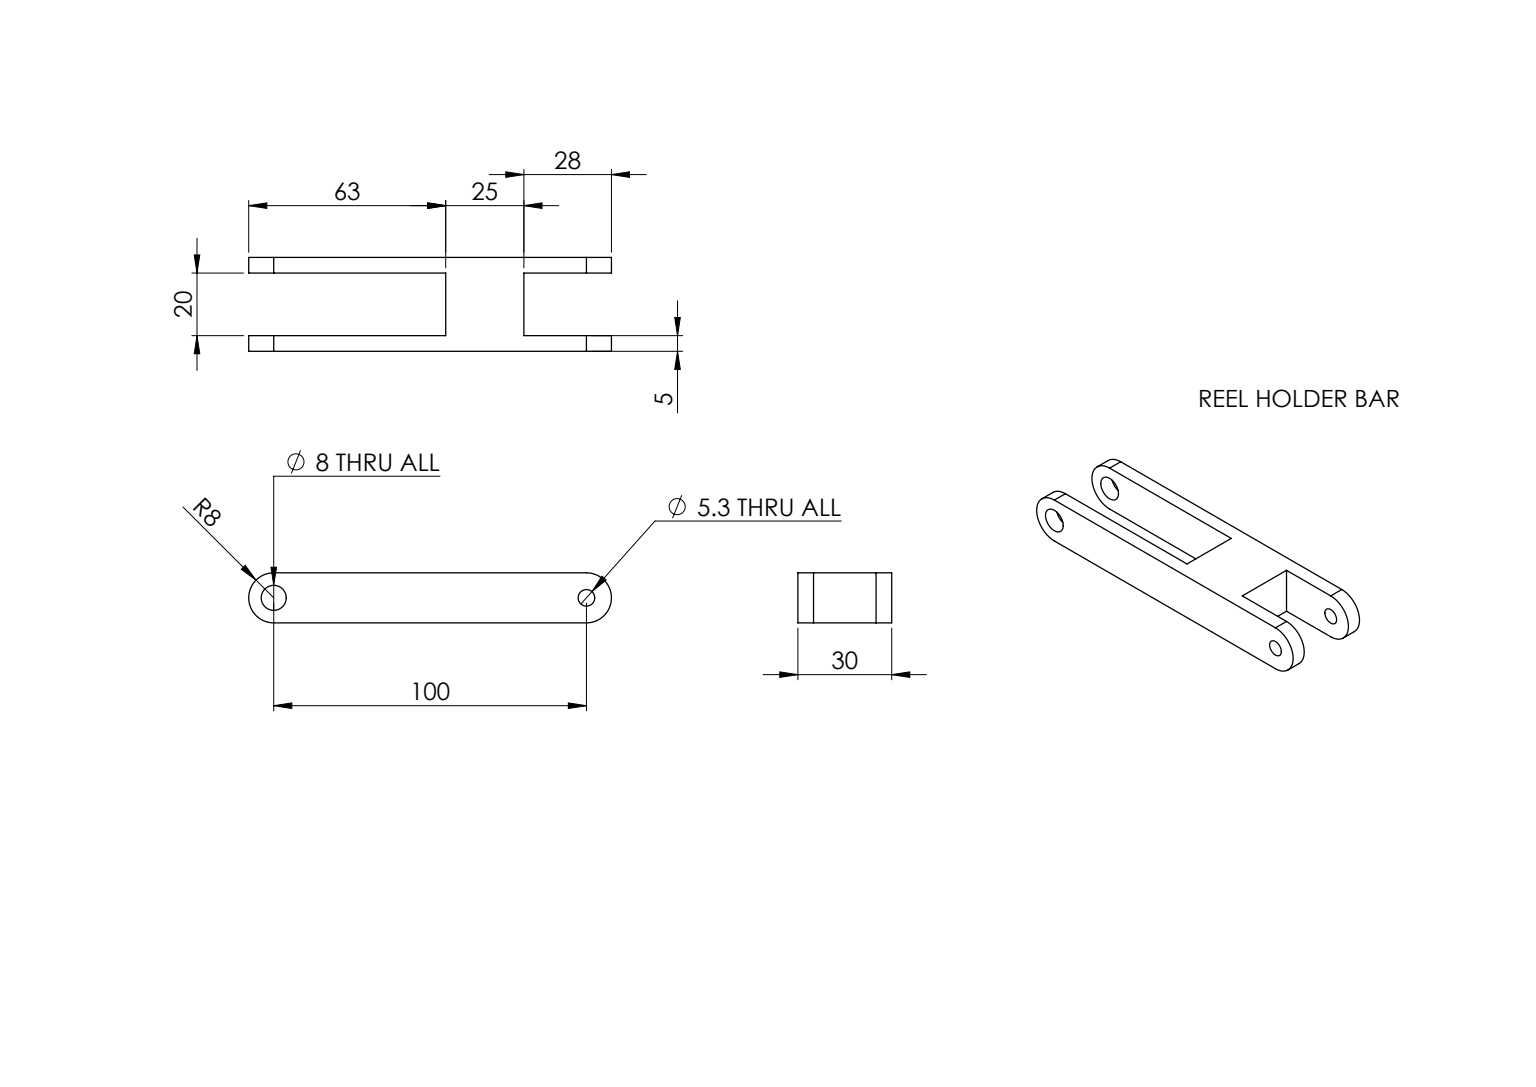
ISO-10303-21;
HEADER;
FILE_DESCRIPTION (('STEP AP214'),
    '1' );
FILE_NAME ('reel holder bar.step',
    '2026-10-31T03:44:21',
    ( '' ),
    ( '' ),
    'SwSTEP 2.0',
    'SolidWorks 2026',
    '' );
FILE_SCHEMA (( 'AUTOMOTIVE_DESIGN' ));
ENDSEC;

DATA;
#6=CARTESIAN_POINT ( 'NONE',  ( -154.9999999999999716, -14.99999999999999645, 15.00000000000000000 ) ) ;
#13=CARTESIAN_POINT ( 'NONE',  ( -57.64999999999994884, -14.99999999999998579, -10.00000000000000178 ) ) ;
#16=SHAPE_DEFINITION_REPRESENTATION ( #10384, #4039 ) ;
#36=ORIENTED_EDGE ( 'NONE', *, *, #18632, .T. ) ;
#48=DIRECTION ( 'NONE',  ( 1.000000000000000000, 0.000000000000000000, 0.000000000000000000 ) ) ;
#67=ORIENTED_EDGE ( 'NONE', *, *, #8672, .F. ) ;
#76=EDGE_LOOP ( 'NONE', ( #8568, #3625 ) ) ;
#82=EDGE_CURVE ( 'NONE', #6843, #7000, #17682, .T. ) ;
#90=ORIENTED_EDGE ( 'NONE', *, *, #9609, .F. ) ;
#105=ADVANCED_FACE ( 'NONE', ( #13344 ), #11768, .F. ) ;
#156=CARTESIAN_POINT ( 'NONE',  ( -99.99999999999997158, -23.00000000000000711, 15.00000000000000000 ) ) ;
#187=ORIENTED_EDGE ( 'NONE', *, *, #1986, .T. ) ;
#278=COLOUR_RGB ( '',0.8941176470588234615, 0.8941176470588234615, 0.8941176470588234615 ) ;
#330=LINE ( 'NONE', #424, #19101 ) ;
#343=CARTESIAN_POINT ( 'NONE',  ( -99.99999999999997158, -23.00000000000000711, -15.00000000000000000 ) ) ;
#347=EDGE_CURVE ( 'NONE', #6641, #7321, #477, .T. ) ;
#365=EDGE_LOOP ( 'NONE', ( #11138, #12423, #1460, #7331 ) ) ;
#402=VERTEX_POINT ( 'NONE', #17273 ) ;
#424=CARTESIAN_POINT ( 'NONE',  ( -158.9999999999999716, -14.99999999999999645, 15.00000000000000000 ) ) ;
#445=LINE ( 'NONE', #18307, #3466 ) ;
#477=CIRCLE ( 'NONE', #6723, 2.649999999999985700 ) ;
#506=DIRECTION ( 'NONE',  ( 1.000000000000000000, 0.000000000000000000, -0.000000000000000000 ) ) ;
#507=CARTESIAN_POINT ( 'NONE',  ( -54.99999999999996447, -14.99999999999998579, 15.00000000000000178 ) ) ;
#515=CARTESIAN_POINT ( 'NONE',  ( -54.99999999999996447, -6.999999999999985789, -10.00000000000000000 ) ) ;
#519=DIRECTION ( 'NONE',  ( 1.000000000000000000, 0.000000000000000000, 0.000000000000000000 ) ) ;
#553=CARTESIAN_POINT ( 'NONE',  ( -162.9999999999999716, -14.99999999999999645, 10.00000000000000000 ) ) ;
#580=ORIENTED_EDGE ( 'NONE', *, *, #7614, .F. ) ;
#608=CARTESIAN_POINT ( 'NONE',  ( -54.99999999999996447, -14.99999999999998579, 15.00000000000000000 ) ) ;
#617=DIRECTION ( 'NONE',  ( -0.000000000000000000, -0.000000000000000000, -1.000000000000000000 ) ) ;
#629=PLANE ( 'NONE',  #12484 ) ;
#657=ORIENTED_EDGE ( 'NONE', *, *, #347, .T. ) ;
#698=FACE_BOUND ( 'NONE', #76, .T. ) ;
#701=DIRECTION ( 'NONE',  ( -1.000000000000000000, -1.387778780781445676E-16, 0.000000000000000000 ) ) ;
#718=DIRECTION ( 'NONE',  ( -1.000000000000000000, 0.000000000000000000, 0.000000000000000000 ) ) ;
#729=PLANE ( 'NONE',  #15634 ) ;
#730=VERTEX_POINT ( 'NONE', #1229 ) ;
#775=ORIENTED_EDGE ( 'NONE', *, *, #19061, .T. ) ;
#790=DIRECTION ( 'NONE',  ( 1.000000000000000000, 0.000000000000000000, 0.000000000000000000 ) ) ;
#812=DIRECTION ( 'NONE',  ( -1.000000000000000000, 0.000000000000000000, 0.000000000000000000 ) ) ;
#824=AXIS2_PLACEMENT_3D ( 'NONE', #3051, #9010, #1576 ) ;
#845=CARTESIAN_POINT ( 'NONE',  ( -54.99999999999996447, -6.999999999999985789, 15.00000000000000000 ) ) ;
#866=DIRECTION ( 'NONE',  ( 1.000000000000000000, 0.000000000000000000, -0.000000000000000000 ) ) ;
#923=FACE_BOUND ( 'NONE', #14792, .T. ) ;
#960=EDGE_CURVE ( 'NONE', #12436, #2436, #8867, .T. ) ;
#962=AXIS2_PLACEMENT_3D ( 'NONE', #2262, #11249, #866 ) ;
#971=FACE_OUTER_BOUND ( 'NONE', #8611, .T. ) ;
#974=VECTOR ( 'NONE', #17216, 1000.000000000000000 ) ;
#1019=DIRECTION ( 'NONE',  ( -0.000000000000000000, -0.000000000000000000, -1.000000000000000000 ) ) ;
#1028=EDGE_CURVE ( 'NONE', #7000, #18623, #12094, .T. ) ;
#1069=ADVANCED_FACE ( 'NONE', ( #18387 ), #11190, .F. ) ;
#1074=VECTOR ( 'NONE', #15077, 1000.000000000000000 ) ;
#1081=VECTOR ( 'NONE', #4236, 1000.000000000000000 ) ;
#1102=FACE_OUTER_BOUND ( 'NONE', #5429, .T. ) ;
#1119=MECHANICAL_DESIGN_GEOMETRIC_PRESENTATION_REPRESENTATION('',(#9556),#3023);
#1121=EDGE_CURVE ( 'NONE', #2436, #4796, #6494, .T. ) ;
#1134=LINE ( 'NONE', #11509, #2767 ) ;
#1143=ORIENTED_EDGE ( 'NONE', *, *, #16287, .T. ) ;
#1148=ORIENTED_EDGE ( 'NONE', *, *, #1495, .F. ) ;
#1157=ADVANCED_FACE ( 'NONE', ( #18483 ), #5123, .T. ) ;
#1195=ORIENTED_EDGE ( 'NONE', *, *, #3564, .F. ) ;
#1204=CARTESIAN_POINT ( 'NONE',  ( -154.9999999999999716, -14.99999999999999645, -15.00000000000000000 ) ) ;
#1229=CARTESIAN_POINT ( 'NONE',  ( -158.9999999999999716, -14.99999999999999645, 15.00000000000000000 ) ) ;
#1257=EDGE_CURVE ( 'NONE', #7908, #5389, #9625, .T. ) ;
#1261=CYLINDRICAL_SURFACE ( 'NONE', #6698, 8.000000000000007105 ) ;
#1263=VECTOR ( 'NONE', #13574, 1000.000000000000000 ) ;
#1265=ORIENTED_EDGE ( 'NONE', *, *, #11172, .F. ) ;
#1270=ADVANCED_FACE ( 'NONE', ( #12871 ), #4238, .T. ) ;
#1324=DIRECTION ( 'NONE',  ( -0.000000000000000000, -0.000000000000000000, 1.000000000000000000 ) ) ;
#1375=EDGE_CURVE ( 'NONE', #3962, #17116, #13061, .T. ) ;
#1379=DIRECTION ( 'NONE',  ( -0.000000000000000000, -0.000000000000000000, 1.000000000000000000 ) ) ;
#1415=FACE_OUTER_BOUND ( 'NONE', #16823, .T. ) ;
#1423=DIRECTION ( 'NONE',  ( -0.000000000000000000, -0.000000000000000000, -1.000000000000000000 ) ) ;
#1460=ORIENTED_EDGE ( 'NONE', *, *, #3650, .F. ) ;
#1484=ORIENTED_EDGE ( 'NONE', *, *, #18632, .F. ) ;
#1490=FACE_OUTER_BOUND ( 'NONE', #10666, .T. ) ;
#1495=EDGE_CURVE ( 'NONE', #18325, #13768, #18729, .T. ) ;
#1517=CARTESIAN_POINT ( 'NONE',  ( -99.99999999999997158, -14.99999999999999289, 10.00000000000000000 ) ) ;
#1536=ORIENTED_EDGE ( 'NONE', *, *, #960, .F. ) ;
#1550=DIRECTION ( 'NONE',  ( -1.000000000000000000, 0.000000000000000000, 0.000000000000000000 ) ) ;
#1569=VERTEX_POINT ( 'NONE', #16405 ) ;
#1576=DIRECTION ( 'NONE',  ( 1.000000000000000000, 0.000000000000000000, 0.000000000000000000 ) ) ;
#1584=ORIENTED_EDGE ( 'NONE', *, *, #9029, .F. ) ;
#1597=DIRECTION ( 'NONE',  ( -0.000000000000000000, -0.000000000000000000, 1.000000000000000000 ) ) ;
#1657=CARTESIAN_POINT ( 'NONE',  ( -54.99999999999996447, -22.99999999999998579, -10.00000000000000000 ) ) ;
#1712=CARTESIAN_POINT ( 'NONE',  ( -154.9999999999999716, -14.99999999999999645, 15.00000000000000000 ) ) ;
#1720=ORIENTED_EDGE ( 'NONE', *, *, #9029, .T. ) ;
#1823=AXIS2_PLACEMENT_3D ( 'NONE', #2602, #8645, #14618 ) ;
#1824=ORIENTED_EDGE ( 'NONE', *, *, #9609, .T. ) ;
#1866=CARTESIAN_POINT ( 'NONE',  ( -162.9999999999999716, -14.99999999999999645, -15.00000000000000000 ) ) ;
#1902=CARTESIAN_POINT ( 'NONE',  ( -57.64999999999994884, -14.99999999999998579, -15.00000000000000000 ) ) ;
#1943=LINE ( 'NONE', #6149, #12265 ) ;
#1954=LINE ( 'NONE', #15566, #5039 ) ;
#1966=ORIENTED_EDGE ( 'NONE', *, *, #13563, .F. ) ;
#1978=EDGE_CURVE ( 'NONE', #18325, #2436, #4519, .T. ) ;
#1980=FACE_OUTER_BOUND ( 'NONE', #5303, .T. ) ;
#1986=EDGE_CURVE ( 'NONE', #18910, #3513, #6765, .T. ) ;
#1989=FACE_OUTER_BOUND ( 'NONE', #9536, .T. ) ;
#2003=CARTESIAN_POINT ( 'NONE',  ( -54.99999999999996447, -22.99999999999998579, 10.00000000000000000 ) ) ;
#2061=VECTOR ( 'NONE', #2153, 1000.000000000000000 ) ;
#2064=CARTESIAN_POINT ( 'NONE',  ( -154.9999999999999716, -14.99999999999999645, 10.00000000000000000 ) ) ;
#2087=EDGE_CURVE ( 'NONE', #3513, #12235, #18251, .T. ) ;
#2094=CARTESIAN_POINT ( 'NONE',  ( -52.34999999999998010, -14.99999999999998579, 15.00000000000000000 ) ) ;
#2104=CARTESIAN_POINT ( 'NONE',  ( -54.99999999999996447, -14.99999999999998579, 10.00000000000000000 ) ) ;
#2148=LINE ( 'NONE', #3813, #18089 ) ;
#2153=DIRECTION ( 'NONE',  ( -0.000000000000000000, -0.000000000000000000, 1.000000000000000000 ) ) ;
#2194=DIRECTION ( 'NONE',  ( -0.000000000000000000, -0.000000000000000000, 1.000000000000000000 ) ) ;
#2196=DIRECTION ( 'NONE',  ( -0.000000000000000000, -0.000000000000000000, 1.000000000000000000 ) ) ;
#2218=EDGE_LOOP ( 'NONE', ( #6703, #580, #17337, #12969, #17413, #15960, #6167, #14004, #1484, #17404, #17241, #18551 ) ) ;
#2255=DIRECTION ( 'NONE',  ( -0.000000000000000000, -0.000000000000000000, 1.000000000000000000 ) ) ;
#2262=CARTESIAN_POINT ( 'NONE',  ( -54.99999999999996447, -14.99999999999998579, 10.00000000000000000 ) ) ;
#2264=MANIFOLD_SOLID_BREP ( 'M5 Clearance Hole1', #17769 ) ;
#2329=EDGE_CURVE ( 'NONE', #13768, #4796, #16555, .T. ) ;
#2336=FILL_AREA_STYLE_COLOUR ( '', #278 ) ;
#2385=EDGE_LOOP ( 'NONE', ( #12298, #7289, #7016, #12127 ) ) ;
#2389=DIRECTION ( 'NONE',  ( 1.000000000000000000, 0.000000000000000000, 0.000000000000000000 ) ) ;
#2436=VERTEX_POINT ( 'NONE', #1657 ) ;
#2450=EDGE_CURVE ( 'NONE', #8156, #4950, #1943, .T. ) ;
#2487=VERTEX_POINT ( 'NONE', #553 ) ;
#2498=CYLINDRICAL_SURFACE ( 'NONE', #6385, 8.000000000000007105 ) ;
#2516=ORIENTED_EDGE ( 'NONE', *, *, #8072, .F. ) ;
#2519=EDGE_CURVE ( 'NONE', #5544, #9930, #7883, .T. ) ;
#2525=LINE ( 'NONE', #8374, #5767 ) ;
#2537=CIRCLE ( 'NONE', #18184, 2.649999999999985700 ) ;
#2597=CYLINDRICAL_SURFACE ( 'NONE', #14386, 4.000000000000003553 ) ;
#2602=CARTESIAN_POINT ( 'NONE',  ( -54.99999999999996447, -14.99999999999998579, 10.00000000000000000 ) ) ;
#2605=CARTESIAN_POINT ( 'NONE',  ( -54.99999999999996447, -14.99999999999998579, 10.00000000000000000 ) ) ;
#2611=VERTEX_POINT ( 'NONE', #10119 ) ;
#2614=ORIENTED_EDGE ( 'NONE', *, *, #5937, .F. ) ;
#2737=LINE ( 'NONE', #5658, #15697 ) ;
#2767=VECTOR ( 'NONE', #19296, 1000.000000000000000 ) ;
#2784=DIRECTION ( 'NONE',  ( 1.000000000000000000, 0.000000000000000000, 0.000000000000000000 ) ) ;
#2815=EDGE_CURVE ( 'NONE', #4950, #11986, #12899, .T. ) ;
#2832=DIRECTION ( 'NONE',  ( 0.000000000000000000, 0.000000000000000000, -1.000000000000000000 ) ) ;
#2871=CARTESIAN_POINT ( 'NONE',  ( 0.000000000000000000, 0.000000000000000000, 0.000000000000000000 ) ) ;
#2880=DIRECTION ( 'NONE',  ( -0.000000000000000000, -0.000000000000000000, 1.000000000000000000 ) ) ;
#2988=ORIENTED_EDGE ( 'NONE', *, *, #6675, .F. ) ;
#3018=EDGE_LOOP ( 'NONE', ( #15293, #8632, #3138, #6074 ) ) ;
#3023=( GEOMETRIC_REPRESENTATION_CONTEXT ( 3 ) GLOBAL_UNCERTAINTY_ASSIGNED_CONTEXT ( ( #12448 ) ) GLOBAL_UNIT_ASSIGNED_CONTEXT ( ( #5376, #17448, #3912 ) ) REPRESENTATION_CONTEXT ( 'NONE', 'WORKASPACE' ) );
#3051=CARTESIAN_POINT ( 'NONE',  ( -154.9999999999999716, -14.99999999999999645, -15.00000000000000000 ) ) ;
#3138=ORIENTED_EDGE ( 'NONE', *, *, #1121, .T. ) ;
#3151=CIRCLE ( 'NONE', #11899, 8.000000000000007105 ) ;
#3187=DIRECTION ( 'NONE',  ( -0.000000000000000000, -0.000000000000000000, 1.000000000000000000 ) ) ;
#3254=VERTEX_POINT ( 'NONE', #9838 ) ;
#3260=DIRECTION ( 'NONE',  ( 1.000000000000000000, 0.000000000000000000, 0.000000000000000000 ) ) ;
#3274=DIRECTION ( 'NONE',  ( -1.000000000000000000, 0.000000000000000000, 0.000000000000000000 ) ) ;
#3283=EDGE_CURVE ( 'NONE', #5389, #16193, #2525, .T. ) ;
#3286=AXIS2_PLACEMENT_3D ( 'NONE', #5019, #15506, #11084 ) ;
#3340=CARTESIAN_POINT ( 'NONE',  ( -54.99999999999996447, -6.999999999999985789, 15.00000000000000000 ) ) ;
#3412=CARTESIAN_POINT ( 'NONE',  ( -54.99999999999996447, -6.999999999999985789, -15.00000000000000000 ) ) ;
#3416=( GEOMETRIC_REPRESENTATION_CONTEXT ( 3 ) GLOBAL_UNCERTAINTY_ASSIGNED_CONTEXT ( ( #11848 ) ) GLOBAL_UNIT_ASSIGNED_CONTEXT ( ( #9563, #12709, #12611 ) ) REPRESENTATION_CONTEXT ( 'NONE', 'WORKASPACE' ) );
#3431=ADVANCED_FACE ( 'NONE', ( #14843 ), #7679, .T. ) ;
#3440=AXIS2_PLACEMENT_3D ( 'NONE', #156, #12393, #3488 ) ;
#3448=CARTESIAN_POINT ( 'NONE',  ( -154.9999999999999716, -14.99999999999999645, -10.00000000000000000 ) ) ;
#3466=VECTOR ( 'NONE', #18217, 1000.000000000000000 ) ;
#3488=DIRECTION ( 'NONE',  ( 1.387778780781445676E-16, -1.000000000000000000, 0.000000000000000000 ) ) ;
#3513=VERTEX_POINT ( 'NONE', #11893 ) ;
#3517=ORIENTED_EDGE ( 'NONE', *, *, #9516, .F. ) ;
#3558=VERTEX_POINT ( 'NONE', #18583 ) ;
#3564=EDGE_CURVE ( 'NONE', #7908, #15389, #18289, .T. ) ;
#3625=ORIENTED_EDGE ( 'NONE', *, *, #2815, .T. ) ;
#3629=ORIENTED_EDGE ( 'NONE', *, *, #13705, .F. ) ;
#3650=EDGE_CURVE ( 'NONE', #11034, #2611, #3754, .T. ) ;
#3660=CARTESIAN_POINT ( 'NONE',  ( -154.9999999999999716, -14.99999999999999645, 15.00000000000000000 ) ) ;
#3695=AXIS2_PLACEMENT_3D ( 'NONE', #1204, #8554, #5318 ) ;
#3716=FACE_BOUND ( 'NONE', #13521, .T. ) ;
#3723=CARTESIAN_POINT ( 'NONE',  ( -154.9999999999999716, -14.99999999999999645, 15.00000000000000000 ) ) ;
#3738=ADVANCED_FACE ( 'NONE', ( #17595 ), #2498, .T. ) ;
#3748=CIRCLE ( 'NONE', #14701, 8.000000000000000000 ) ;
#3754=LINE ( 'NONE', #9913, #1081 ) ;
#3789=CIRCLE ( 'NONE', #10979, 4.000000000000003553 ) ;
#3813=CARTESIAN_POINT ( 'NONE',  ( -154.9999999999999716, -6.999999999999993783, -15.00000000000000000 ) ) ;
#3850=CARTESIAN_POINT ( 'NONE',  ( -99.99999999999997158, -23.00000000000000711, -10.00000000000000178 ) ) ;
#3868=ORIENTED_EDGE ( 'NONE', *, *, #9565, .F. ) ;
#3895=SURFACE_SIDE_STYLE ('',( #5067 ) ) ;
#3912=( NAMED_UNIT ( * ) SI_UNIT ( $, .STERADIAN. ) SOLID_ANGLE_UNIT ( ) );
#3926=ORIENTED_EDGE ( 'NONE', *, *, #18352, .T. ) ;
#3955=DIRECTION ( 'NONE',  ( 1.000000000000000000, 0.000000000000000000, 0.000000000000000000 ) ) ;
#3962=VERTEX_POINT ( 'NONE', #13639 ) ;
#3964=ORIENTED_EDGE ( 'NONE', *, *, #2815, .F. ) ;
#4009=ADVANCED_FACE ( 'NONE', ( #1980, #698 ), #16787, .F. ) ;
#4039=SHAPE_REPRESENTATION ( 'reel holder bar', ( #10359 ), #3416 ) ;
#4132=ADVANCED_FACE ( 'NONE', ( #13733 ), #4822, .F. ) ;
#4164=LINE ( 'NONE', #11498, #974 ) ;
#4229=EDGE_CURVE ( 'NONE', #402, #17786, #9698, .T. ) ;
#4233=DIRECTION ( 'NONE',  ( -0.000000000000000000, -0.000000000000000000, 1.000000000000000000 ) ) ;
#4236=DIRECTION ( 'NONE',  ( 0.000000000000000000, 0.000000000000000000, -1.000000000000000000 ) ) ;
#4238=CYLINDRICAL_SURFACE ( 'NONE', #3695, 8.000000000000007105 ) ;
#4246=VECTOR ( 'NONE', #19233, 1000.000000000000000 ) ;
#4272=DIRECTION ( 'NONE',  ( 1.000000000000000000, 1.387778780781445676E-16, -0.000000000000000000 ) ) ;
#4308=ORIENTED_EDGE ( 'NONE', *, *, #18352, .F. ) ;
#4334=CARTESIAN_POINT ( 'NONE',  ( -154.9999999999999716, -23.00000000000000000, 15.00000000000000000 ) ) ;
#4373=EDGE_CURVE ( 'NONE', #1569, #6843, #5468, .T. ) ;
#4405=LINE ( 'NONE', #13220, #15601 ) ;
#4443=DIRECTION ( 'NONE',  ( -0.000000000000000000, -0.000000000000000000, -1.000000000000000000 ) ) ;
#4467=DIRECTION ( 'NONE',  ( 0.000000000000000000, 0.000000000000000000, -1.000000000000000000 ) ) ;
#4519=LINE ( 'NONE', #13621, #17110 ) ;
#4553=CARTESIAN_POINT ( 'NONE',  ( -54.99999999999996447, -6.999999999999985789, 15.00000000000000000 ) ) ;
#4610=DIRECTION ( 'NONE',  ( 1.000000000000000000, 0.000000000000000000, 0.000000000000000000 ) ) ;
#4612=VECTOR ( 'NONE', #4443, 1000.000000000000000 ) ;
#4643=VECTOR ( 'NONE', #5032, 1000.000000000000000 ) ;
#4645=ORIENTED_EDGE ( 'NONE', *, *, #19255, .F. ) ;
#4654=ORIENTED_EDGE ( 'NONE', *, *, #18569, .T. ) ;
#4659=CIRCLE ( 'NONE', #12459, 4.000000000000003553 ) ;
#4662=FACE_BOUND ( 'NONE', #6040, .T. ) ;
#4691=LINE ( 'NONE', #11193, #1074 ) ;
#4701=VERTEX_POINT ( 'NONE', #17544 ) ;
#4706=ORIENTED_EDGE ( 'NONE', *, *, #10750, .F. ) ;
#4721=VECTOR ( 'NONE', #8042, 1000.000000000000000 ) ;
#4796=VERTEX_POINT ( 'NONE', #15674 ) ;
#4819=CYLINDRICAL_SURFACE ( 'NONE', #7205, 2.649999999999985700 ) ;
#4822=CYLINDRICAL_SURFACE ( 'NONE', #4833, 2.649999999999985700 ) ;
#4833=AXIS2_PLACEMENT_3D ( 'NONE', #10983, #16990, #15491 ) ;
#4859=PLANE ( 'NONE',  #3440 ) ;
#4907=DIRECTION ( 'NONE',  ( 1.000000000000000000, 0.000000000000000000, 0.000000000000000000 ) ) ;
#4920=CYLINDRICAL_SURFACE ( 'NONE', #16636, 2.649999999999985700 ) ;
#4941=EDGE_LOOP ( 'NONE', ( #1584, #8466, #13261, #15641 ) ) ;
#4950=VERTEX_POINT ( 'NONE', #16457 ) ;
#4954=ADVANCED_FACE ( 'NONE', ( #10452 ), #1261, .T. ) ;
#4996=LINE ( 'NONE', #17461, #4246 ) ;
#5019=CARTESIAN_POINT ( 'NONE',  ( -154.9999999999999716, -14.99999999999999645, 10.00000000000000000 ) ) ;
#5020=EDGE_CURVE ( 'NONE', #8949, #17786, #4691, .T. ) ;
#5032=DIRECTION ( 'NONE',  ( 1.000000000000000000, 1.387778780781445676E-16, -0.000000000000000000 ) ) ;
#5039=VECTOR ( 'NONE', #2255, 1000.000000000000000 ) ;
#5064=ORIENTED_EDGE ( 'NONE', *, *, #8672, .T. ) ;
#5067=SURFACE_STYLE_FILL_AREA ( #17339 ) ;
#5123=CYLINDRICAL_SURFACE ( 'NONE', #15589, 8.000000000000007105 ) ;
#5135=DIRECTION ( 'NONE',  ( -1.387778780781445676E-16, 1.000000000000000000, 0.000000000000000000 ) ) ;
#5163=ORIENTED_EDGE ( 'NONE', *, *, #18080, .T. ) ;
#5191=EDGE_CURVE ( 'NONE', #13489, #7050, #5772, .T. ) ;
#5195=EDGE_CURVE ( 'NONE', #3513, #13956, #11379, .T. ) ;
#5215=DIRECTION ( 'NONE',  ( -0.000000000000000000, -0.000000000000000000, -1.000000000000000000 ) ) ;
#5303=EDGE_LOOP ( 'NONE', ( #8693, #15482, #775, #19219, #8129 ) ) ;
#5306=EDGE_CURVE ( 'NONE', #1569, #2487, #13161, .T. ) ;
#5318=DIRECTION ( 'NONE',  ( -1.000000000000000000, 0.000000000000000000, 0.000000000000000000 ) ) ;
#5325=CARTESIAN_POINT ( 'NONE',  ( -154.9999999999999716, -6.999999999999993783, -15.00000000000000000 ) ) ;
#5358=ORIENTED_EDGE ( 'NONE', *, *, #12392, .T. ) ;
#5360=ORIENTED_EDGE ( 'NONE', *, *, #6450, .T. ) ;
#5376=( LENGTH_UNIT ( ) NAMED_UNIT ( * ) SI_UNIT ( .MILLI., .METRE. ) );
#5389=VERTEX_POINT ( 'NONE', #15119 ) ;
#5414=DIRECTION ( 'NONE',  ( 0.000000000000000000, 0.000000000000000000, 1.000000000000000000 ) ) ;
#5422=DIRECTION ( 'NONE',  ( 0.000000000000000000, 0.000000000000000000, 1.000000000000000000 ) ) ;
#5429=EDGE_LOOP ( 'NONE', ( #17900, #11793, #10748, #67 ) ) ;
#5459=ORIENTED_EDGE ( 'NONE', *, *, #18569, .F. ) ;
#5468=CIRCLE ( 'NONE', #16766, 8.000000000000007105 ) ;
#5530=AXIS2_PLACEMENT_3D ( 'NONE', #17774, #8935, #10300 ) ;
#5544=VERTEX_POINT ( 'NONE', #10699 ) ;
#5648=EDGE_LOOP ( 'NONE', ( #14542, #2614 ) ) ;
#5658=CARTESIAN_POINT ( 'NONE',  ( -154.9999999999999716, -23.00000000000000000, -15.00000000000000000 ) ) ;
#5664=AXIS2_PLACEMENT_3D ( 'NONE', #16412, #9039, #7186 ) ;
#5667=ADVANCED_FACE ( 'NONE', ( #9420 ), #7947, .F. ) ;
#5681=DIRECTION ( 'NONE',  ( -1.000000000000000000, 0.000000000000000000, 0.000000000000000000 ) ) ;
#5712=CARTESIAN_POINT ( 'NONE',  ( -74.99999999999997158, -22.99999999999998934, -10.00000000000000000 ) ) ;
#5767=VECTOR ( 'NONE', #8481, 1000.000000000000000 ) ;
#5772=CIRCLE ( 'NONE', #6374, 8.000000000000000000 ) ;
#5775=DIRECTION ( 'NONE',  ( -1.000000000000000000, -1.040834085586084257E-16, -0.000000000000000000 ) ) ;
#5777=CARTESIAN_POINT ( 'NONE',  ( -54.99999999999996447, -14.99999999999998579, -10.00000000000000178 ) ) ;
#5780=EDGE_LOOP ( 'NONE', ( #657, #1824 ) ) ;
#5810=DIRECTION ( 'NONE',  ( -0.000000000000000000, -0.000000000000000000, 1.000000000000000000 ) ) ;
#5838=DIRECTION ( 'NONE',  ( 0.000000000000000000, 0.000000000000000000, -1.000000000000000000 ) ) ;
#5849=ORIENTED_EDGE ( 'NONE', *, *, #12619, .T. ) ;
#5856=DIRECTION ( 'NONE',  ( -1.000000000000000000, 0.000000000000000000, 0.000000000000000000 ) ) ;
#5915=( GEOMETRIC_REPRESENTATION_CONTEXT ( 3 ) GLOBAL_UNCERTAINTY_ASSIGNED_CONTEXT ( ( #12427 ) ) GLOBAL_UNIT_ASSIGNED_CONTEXT ( ( #15851, #18812, #16948 ) ) REPRESENTATION_CONTEXT ( 'NONE', 'WORKASPACE' ) );
#5930=ORIENTED_EDGE ( 'NONE', *, *, #11172, .T. ) ;
#5937=EDGE_CURVE ( 'NONE', #16193, #15389, #15991, .T. ) ;
#5950=CIRCLE ( 'NONE', #10621, 2.649999999999985700 ) ;
#5970=VERTEX_POINT ( 'NONE', #11752 ) ;
#5984=EDGE_CURVE ( 'NONE', #2487, #7000, #17877, .T. ) ;
#6031=DIRECTION ( 'NONE',  ( 1.387778780781445676E-16, -1.000000000000000000, 0.000000000000000000 ) ) ;
#6040=EDGE_LOOP ( 'NONE', ( #5360, #15655 ) ) ;
#6074=ORIENTED_EDGE ( 'NONE', *, *, #7614, .T. ) ;
#6116=DIRECTION ( 'NONE',  ( 1.000000000000000000, 0.000000000000000000, 0.000000000000000000 ) ) ;
#6123=CARTESIAN_POINT ( 'NONE',  ( -54.99999999999996447, -22.99999999999998579, -10.00000000000000000 ) ) ;
#6126=AXIS2_PLACEMENT_3D ( 'NONE', #3723, #14300, #4907 ) ;
#6128=CARTESIAN_POINT ( 'NONE',  ( -54.99999999999996447, -6.999999999999985789, 10.00000000000000000 ) ) ;
#6149=CARTESIAN_POINT ( 'NONE',  ( -158.9999999999999716, -14.99999999999999645, 15.00000000000000000 ) ) ;
#6167=ORIENTED_EDGE ( 'NONE', *, *, #13705, .T. ) ;
#6203=CARTESIAN_POINT ( 'NONE',  ( -54.99999999999996447, -22.99999999999998579, 15.00000000000000000 ) ) ;
#6212=LINE ( 'NONE', #1517, #7714 ) ;
#6277=ORIENTED_EDGE ( 'NONE', *, *, #5984, .F. ) ;
#6278=ADVANCED_FACE ( 'NONE', ( #3716, #971 ), #17354, .F. ) ;
#6294=DIRECTION ( 'NONE',  ( 0.000000000000000000, 0.000000000000000000, -1.000000000000000000 ) ) ;
#6303=PLANE ( 'NONE',  #9311 ) ;
#6318=PLANE ( 'NONE',  #12056 ) ;
#6348=DIRECTION ( 'NONE',  ( -0.000000000000000000, -0.000000000000000000, 1.000000000000000000 ) ) ;
#6374=AXIS2_PLACEMENT_3D ( 'NONE', #2605, #5414, #3955 ) ;
#6383=DIRECTION ( 'NONE',  ( 1.000000000000000000, 0.000000000000000000, 0.000000000000000000 ) ) ;
#6385=AXIS2_PLACEMENT_3D ( 'NONE', #7076, #19068, #812 ) ;
#6390=DIRECTION ( 'NONE',  ( -0.000000000000000000, -0.000000000000000000, 1.000000000000000000 ) ) ;
#6450=EDGE_CURVE ( 'NONE', #14431, #8156, #3789, .T. ) ;
#6468=CARTESIAN_POINT ( 'NONE',  ( -54.99999999999996447, -14.99999999999998579, -10.00000000000000000 ) ) ;
#6494=CIRCLE ( 'NONE', #14637, 8.000000000000000000 ) ;
#6524=DIRECTION ( 'NONE',  ( 0.000000000000000000, 0.000000000000000000, 1.000000000000000000 ) ) ;
#6531=PRESENTATION_STYLE_ASSIGNMENT (( #17137 ) ) ;
#6583=FACE_OUTER_BOUND ( 'NONE', #3018, .T. ) ;
#6641=VERTEX_POINT ( 'NONE', #9945 ) ;
#6647=DIRECTION ( 'NONE',  ( -0.000000000000000000, -0.000000000000000000, 1.000000000000000000 ) ) ;
#6656=ORIENTED_EDGE ( 'NONE', *, *, #16120, .F. ) ;
#6675=EDGE_CURVE ( 'NONE', #10827, #7050, #12604, .T. ) ;
#6687=FACE_OUTER_BOUND ( 'NONE', #15827, .T. ) ;
#6698=AXIS2_PLACEMENT_3D ( 'NONE', #11982, #17647, #1550 ) ;
#6702=DIRECTION ( 'NONE',  ( 1.000000000000000000, 1.387778780781445676E-16, 0.000000000000000000 ) ) ;
#6703=ORIENTED_EDGE ( 'NONE', *, *, #3650, .T. ) ;
#6705=EDGE_LOOP ( 'NONE', ( #6656, #19117, #12616, #5163 ) ) ;
#6723=AXIS2_PLACEMENT_3D ( 'NONE', #11262, #15696, #7053 ) ;
#6758=DIRECTION ( 'NONE',  ( -0.000000000000000000, -0.000000000000000000, 1.000000000000000000 ) ) ;
#6765=CIRCLE ( 'NONE', #824, 8.000000000000007105 ) ;
#6778=PLANE ( 'NONE',  #8756 ) ;
#6819=DIRECTION ( 'NONE',  ( -0.000000000000000000, -0.000000000000000000, -1.000000000000000000 ) ) ;
#6843=VERTEX_POINT ( 'NONE', #14947 ) ;
#6848=EDGE_LOOP ( 'NONE', ( #12257, #7527, #15829, #13603 ) ) ;
#6882=VECTOR ( 'NONE', #4272, 1000.000000000000000 ) ;
#6883=EDGE_CURVE ( 'NONE', #11986, #4950, #9731, .T. ) ;
#6896=CARTESIAN_POINT ( 'NONE',  ( -74.99999999999997158, -23.00000000000000355, 15.00000000000000000 ) ) ;
#7000=VERTEX_POINT ( 'NONE', #11011 ) ;
#7016=ORIENTED_EDGE ( 'NONE', *, *, #3564, .T. ) ;
#7050=VERTEX_POINT ( 'NONE', #6128 ) ;
#7053=DIRECTION ( 'NONE',  ( -1.000000000000000000, 0.000000000000000000, 0.000000000000000000 ) ) ;
#7076=CARTESIAN_POINT ( 'NONE',  ( -154.9999999999999716, -14.99999999999999645, -15.00000000000000000 ) ) ;
#7112=LINE ( 'NONE', #11617, #15979 ) ;
#7123=ORIENTED_EDGE ( 'NONE', *, *, #2450, .F. ) ;
#7141=AXIS2_PLACEMENT_3D ( 'NONE', #3660, #2196, #17101 ) ;
#7146=LINE ( 'NONE', #9880, #10864 ) ;
#7164=CARTESIAN_POINT ( 'NONE',  ( -154.9999999999999716, -14.99999999999999645, 15.00000000000000000 ) ) ;
#7171=EDGE_CURVE ( 'NONE', #12831, #13489, #9628, .T. ) ;
#7179=DIRECTION ( 'NONE',  ( -1.000000000000000000, -1.040834085586084257E-16, 0.000000000000000000 ) ) ;
#7186=DIRECTION ( 'NONE',  ( 1.000000000000000000, 0.000000000000000000, 0.000000000000000000 ) ) ;
#7205=AXIS2_PLACEMENT_3D ( 'NONE', #10783, #16785, #9313 ) ;
#7281=DIRECTION ( 'NONE',  ( 1.000000000000000000, 0.000000000000000000, 0.000000000000000000 ) ) ;
#7289=ORIENTED_EDGE ( 'NONE', *, *, #1257, .F. ) ;
#7312=ORIENTED_EDGE ( 'NONE', *, *, #18047, .T. ) ;
#7321=VERTEX_POINT ( 'NONE', #13 ) ;
#7331=ORIENTED_EDGE ( 'NONE', *, *, #12619, .F. ) ;
#7342=EDGE_LOOP ( 'NONE', ( #16954, #1148, #3926, #12086, #9214 ) ) ;
#7350=EDGE_CURVE ( 'NONE', #8156, #14431, #11776, .T. ) ;
#7353=DIRECTION ( 'NONE',  ( 0.000000000000000000, 0.000000000000000000, 1.000000000000000000 ) ) ;
#7370=EDGE_CURVE ( 'NONE', #3962, #18623, #6212, .T. ) ;
#7389=DIRECTION ( 'NONE',  ( -1.387778780781445676E-16, 1.000000000000000000, 0.000000000000000000 ) ) ;
#7391=CARTESIAN_POINT ( 'NONE',  ( -99.99999999999997158, -23.00000000000000711, 15.00000000000000000 ) ) ;
#7510=AXIS2_PLACEMENT_3D ( 'NONE', #7164, #8830, #13144 ) ;
#7527=ORIENTED_EDGE ( 'NONE', *, *, #5306, .T. ) ;
#7578=CARTESIAN_POINT ( 'NONE',  ( -57.64999999999994884, -14.99999999999998579, 15.00000000000000178 ) ) ;
#7595=CARTESIAN_POINT ( 'NONE',  ( -99.99999999999997158, -22.99999999999999289, 10.00000000000000000 ) ) ;
#7614=EDGE_CURVE ( 'NONE', #4796, #2611, #15613, .T. ) ;
#7656=ADVANCED_FACE ( 'NONE', ( #6687 ), #13934, .T. ) ;
#7679=CYLINDRICAL_SURFACE ( 'NONE', #10136, 8.000000000000007105 ) ;
#7714=VECTOR ( 'NONE', #6031, 1000.000000000000000 ) ;
#7779=CIRCLE ( 'NONE', #10263, 2.649999999999985700 ) ;
#7846=CIRCLE ( 'NONE', #15360, 2.649999999999985700 ) ;
#7876=EDGE_CURVE ( 'NONE', #13768, #18910, #13616, .T. ) ;
#7883=CIRCLE ( 'NONE', #13519, 4.000000000000003553 ) ;
#7895=ORIENTED_EDGE ( 'NONE', *, *, #9516, .T. ) ;
#7908=VERTEX_POINT ( 'NONE', #15281 ) ;
#7916=ORIENTED_EDGE ( 'NONE', *, *, #5306, .F. ) ;
#7920=CARTESIAN_POINT ( 'NONE',  ( -154.9999999999999716, -14.99999999999999645, -15.00000000000000000 ) ) ;
#7929=DIRECTION ( 'NONE',  ( 1.040834085586084257E-16, -1.000000000000000000, 0.000000000000000000 ) ) ;
#7947=PLANE ( 'NONE',  #18548 ) ;
#8000=SHAPE_REPRESENTATION_RELATIONSHIP ( 'NONE' , 'NONE' ,  #4039, #14807 ) ;
#8017=DIRECTION ( 'NONE',  ( 1.000000000000000000, 0.000000000000000000, 0.000000000000000000 ) ) ;
#8021=PLANE ( 'NONE',  #11835 ) ;
#8026=DIRECTION ( 'NONE',  ( 0.000000000000000000, 0.000000000000000000, 1.000000000000000000 ) ) ;
#8042=DIRECTION ( 'NONE',  ( 1.000000000000000000, 1.387778780781445676E-16, -0.000000000000000000 ) ) ;
#8070=FACE_BOUND ( 'NONE', #5648, .T. ) ;
#8072=EDGE_CURVE ( 'NONE', #18910, #4701, #2148, .T. ) ;
#8129=ORIENTED_EDGE ( 'NONE', *, *, #5020, .T. ) ;
#8156=VERTEX_POINT ( 'NONE', #12625 ) ;
#8157=DIRECTION ( 'NONE',  ( -1.000000000000000000, 0.000000000000000000, 0.000000000000000000 ) ) ;
#8172=CARTESIAN_POINT ( 'NONE',  ( -54.99999999999996447, -14.99999999999998579, 15.00000000000000000 ) ) ;
#8360=AXIS2_PLACEMENT_3D ( 'NONE', #8841, #17681, #19170 ) ;
#8374=CARTESIAN_POINT ( 'NONE',  ( -57.64999999999994884, -14.99999999999998579, 15.00000000000000000 ) ) ;
#8426=CARTESIAN_POINT ( 'NONE',  ( -99.99999999999997158, -23.00000000000000711, -10.00000000000000178 ) ) ;
#8442=ORIENTED_EDGE ( 'NONE', *, *, #16287, .F. ) ;
#8466=ORIENTED_EDGE ( 'NONE', *, *, #16120, .T. ) ;
#8481=DIRECTION ( 'NONE',  ( -0.000000000000000000, -0.000000000000000000, 1.000000000000000000 ) ) ;
#8512=ORIENTED_EDGE ( 'NONE', *, *, #1028, .F. ) ;
#8521=ORIENTED_EDGE ( 'NONE', *, *, #1375, .F. ) ;
#8554=DIRECTION ( 'NONE',  ( -0.000000000000000000, -0.000000000000000000, 1.000000000000000000 ) ) ;
#8564=ORIENTED_EDGE ( 'NONE', *, *, #10750, .T. ) ;
#8568=ORIENTED_EDGE ( 'NONE', *, *, #6883, .T. ) ;
#8585=DIRECTION ( 'NONE',  ( -1.000000000000000000, -1.387778780781445182E-16, -0.000000000000000000 ) ) ;
#8611=EDGE_LOOP ( 'NONE', ( #5459, #5849, #3868, #9281 ) ) ;
#8632=ORIENTED_EDGE ( 'NONE', *, *, #960, .T. ) ;
#8645=DIRECTION ( 'NONE',  ( 0.000000000000000000, 0.000000000000000000, 1.000000000000000000 ) ) ;
#8672=EDGE_CURVE ( 'NONE', #14431, #11986, #1134, .T. ) ;
#8681=ORIENTED_EDGE ( 'NONE', *, *, #1028, .T. ) ;
#8693=ORIENTED_EDGE ( 'NONE', *, *, #4229, .F. ) ;
#8756=AXIS2_PLACEMENT_3D ( 'NONE', #12569, #15807, #11085 ) ;
#8792=VECTOR ( 'NONE', #6819, 1000.000000000000000 ) ;
#8796=ADVANCED_FACE ( 'NONE', ( #12291, #18100, #4662 ), #6318, .T. ) ;
#8830=DIRECTION ( 'NONE',  ( -0.000000000000000000, -0.000000000000000000, 1.000000000000000000 ) ) ;
#8834=DIRECTION ( 'NONE',  ( 0.000000000000000000, 0.000000000000000000, 1.000000000000000000 ) ) ;
#8841=CARTESIAN_POINT ( 'NONE',  ( -154.9999999999999716, -14.99999999999999645, 15.00000000000000000 ) ) ;
#8860=LINE ( 'NONE', #7391, #18208 ) ;
#8867=LINE ( 'NONE', #6123, #10086 ) ;
#8919=CARTESIAN_POINT ( 'NONE',  ( -54.99999999999996447, -14.99999999999998579, 15.00000000000000178 ) ) ;
#8935=DIRECTION ( 'NONE',  ( -0.000000000000000000, -0.000000000000000000, 1.000000000000000000 ) ) ;
#8949=VERTEX_POINT ( 'NONE', #17721 ) ;
#8994=CARTESIAN_POINT ( 'NONE',  ( -54.99999999999996447, -22.99999999999998579, 10.00000000000000000 ) ) ;
#9010=DIRECTION ( 'NONE',  ( -0.000000000000000000, -0.000000000000000000, 1.000000000000000000 ) ) ;
#9029=EDGE_CURVE ( 'NONE', #9930, #5544, #14868, .T. ) ;
#9039=DIRECTION ( 'NONE',  ( -0.000000000000000000, -0.000000000000000000, 1.000000000000000000 ) ) ;
#9048=VECTOR ( 'NONE', #7389, 1000.000000000000000 ) ;
#9214=ORIENTED_EDGE ( 'NONE', *, *, #1986, .F. ) ;
#9281=ORIENTED_EDGE ( 'NONE', *, *, #5191, .F. ) ;
#9311=AXIS2_PLACEMENT_3D ( 'NONE', #12276, #13920, #506 ) ;
#9313=DIRECTION ( 'NONE',  ( 1.000000000000000000, 0.000000000000000000, 0.000000000000000000 ) ) ;
#9343=DIRECTION ( 'NONE',  ( 0.000000000000000000, 0.000000000000000000, 1.000000000000000000 ) ) ;
#9365=CARTESIAN_POINT ( 'NONE',  ( -154.9999999999999716, -14.99999999999999645, 10.00000000000000000 ) ) ;
#9395=ADVANCED_FACE ( 'NONE', ( #18360 ), #11156, .F. ) ;
#9406=ORIENTED_EDGE ( 'NONE', *, *, #12392, .F. ) ;
#9420=FACE_OUTER_BOUND ( 'NONE', #12137, .T. ) ;
#9472=CARTESIAN_POINT ( 'NONE',  ( -154.9999999999999716, -6.999999999999993783, 15.00000000000000000 ) ) ;
#9489=ORIENTED_EDGE ( 'NONE', *, *, #3283, .T. ) ;
#9513=LINE ( 'NONE', #6203, #4721 ) ;
#9516=EDGE_CURVE ( 'NONE', #17116, #2487, #12696, .T. ) ;
#9536=EDGE_LOOP ( 'NONE', ( #8521, #10640, #8512, #6277, #3517 ) ) ;
#9542=EDGE_LOOP ( 'NONE', ( #4706, #9548, #17796, #90 ) ) ;
#9548=ORIENTED_EDGE ( 'NONE', *, *, #18047, .F. ) ;
#9556=STYLED_ITEM('',(#19454),#2264);
#9563=( LENGTH_UNIT ( ) NAMED_UNIT ( * ) SI_UNIT ( .MILLI., .METRE. ) );
#9565=EDGE_CURVE ( 'NONE', #7050, #11034, #4996, .T. ) ;
#9609=EDGE_CURVE ( 'NONE', #7321, #6641, #13009, .T. ) ;
#9613=CARTESIAN_POINT ( 'NONE',  ( -74.99999999999997158, -6.999999999999989342, 10.00000000000000000 ) ) ;
#9625=CIRCLE ( 'NONE', #1823, 2.649999999999985700 ) ;
#9628=LINE ( 'NONE', #14443, #12861 ) ;
#9646=APPLICATION_CONTEXT ( 'automotive_design' ) ;
#9698=LINE ( 'NONE', #8426, #12037 ) ;
#9731=CIRCLE ( 'NONE', #16651, 4.000000000000003553 ) ;
#9738=CARTESIAN_POINT ( 'NONE',  ( -74.99999999999997158, -23.00000000000000355, -10.00000000000000178 ) ) ;
#9808=FACE_BOUND ( 'NONE', #5780, .T. ) ;
#9838=CARTESIAN_POINT ( 'NONE',  ( -74.99999999999997158, -23.00000000000000355, 10.00000000000000000 ) ) ;
#9880=CARTESIAN_POINT ( 'NONE',  ( -74.99999999999997158, -14.99999999999998934, 10.00000000000000000 ) ) ;
#9913=CARTESIAN_POINT ( 'NONE',  ( -74.99999999999997158, -6.999999999999989342, 15.00000000000000000 ) ) ;
#9930=VERTEX_POINT ( 'NONE', #13977 ) ;
#9945=CARTESIAN_POINT ( 'NONE',  ( -52.34999999999998010, -14.99999999999998579, -10.00000000000000178 ) ) ;
#10086=VECTOR ( 'NONE', #14847, 1000.000000000000000 ) ;
#10119=CARTESIAN_POINT ( 'NONE',  ( -74.99999999999997158, -6.999999999999989342, -10.00000000000000178 ) ) ;
#10136=AXIS2_PLACEMENT_3D ( 'NONE', #1712, #1423, #3274 ) ;
#10160=CARTESIAN_POINT ( 'NONE',  ( -154.9999999999999716, -14.99999999999999645, -10.00000000000000178 ) ) ;
#10204=AXIS2_PLACEMENT_3D ( 'NONE', #18479, #5215, #8157 ) ;
#10209=PRODUCT_DEFINITION ( 'UNKNOWN', '', #14488, #13426 ) ;
#10211=EDGE_CURVE ( 'NONE', #3558, #6641, #13103, .T. ) ;
#10221=CYLINDRICAL_SURFACE ( 'NONE', #19152, 4.000000000000003553 ) ;
#10247=ORIENTED_EDGE ( 'NONE', *, *, #2519, .T. ) ;
#10263=AXIS2_PLACEMENT_3D ( 'NONE', #19253, #16395, #16295 ) ;
#10300=DIRECTION ( 'NONE',  ( 1.000000000000000000, 0.000000000000000000, 0.000000000000000000 ) ) ;
#10336=ORIENTED_EDGE ( 'NONE', *, *, #12551, .F. ) ;
#10339=ORIENTED_EDGE ( 'NONE', *, *, #2087, .F. ) ;
#10359=AXIS2_PLACEMENT_3D ( 'NONE', #2871, #8834, #16191 ) ;
#10384=PRODUCT_DEFINITION_SHAPE ( 'NONE', 'NONE',  #10209 ) ;
#10452=FACE_OUTER_BOUND ( 'NONE', #11212, .T. ) ;
#10484=DIRECTION ( 'NONE',  ( -0.000000000000000000, -0.000000000000000000, 1.000000000000000000 ) ) ;
#10573=DIRECTION ( 'NONE',  ( -0.000000000000000000, -0.000000000000000000, 1.000000000000000000 ) ) ;
#10577=EDGE_CURVE ( 'NONE', #10827, #13823, #445, .T. ) ;
#10621=AXIS2_PLACEMENT_3D ( 'NONE', #11677, #4233, #17680 ) ;
#10625=LINE ( 'NONE', #18008, #6882 ) ;
#10640=ORIENTED_EDGE ( 'NONE', *, *, #7370, .T. ) ;
#10666=EDGE_LOOP ( 'NONE', ( #18244, #9489, #18144, #1195 ) ) ;
#10699=CARTESIAN_POINT ( 'NONE',  ( -150.9999999999999716, -14.99999999999999645, 10.00000000000000000 ) ) ;
#10748=ORIENTED_EDGE ( 'NONE', *, *, #6883, .F. ) ;
#10750=EDGE_CURVE ( 'NONE', #17750, #7321, #4164, .T. ) ;
#10759=ORIENTED_EDGE ( 'NONE', *, *, #7370, .F. ) ;
#10783=CARTESIAN_POINT ( 'NONE',  ( -54.99999999999996447, -14.99999999999998579, 15.00000000000000000 ) ) ;
#10815=ADVANCED_FACE ( 'NONE', ( #1415 ), #10221, .F. ) ;
#10827=VERTEX_POINT ( 'NONE', #4553 ) ;
#10864=VECTOR ( 'NONE', #13124, 1000.000000000000000 ) ;
#10877=AXIS2_PLACEMENT_3D ( 'NONE', #15018, #1597, #3260 ) ;
#10885=DIRECTION ( 'NONE',  ( -1.387778780781445676E-16, 1.000000000000000000, 0.000000000000000000 ) ) ;
#10914=ORIENTED_EDGE ( 'NONE', *, *, #10960, .T. ) ;
#10939=CIRCLE ( 'NONE', #7510, 4.000000000000003553 ) ;
#10960=EDGE_CURVE ( 'NONE', #17786, #18623, #8860, .T. ) ;
#10979=AXIS2_PLACEMENT_3D ( 'NONE', #7920, #12030, #13214 ) ;
#10983=CARTESIAN_POINT ( 'NONE',  ( -54.99999999999996447, -14.99999999999998579, 15.00000000000000000 ) ) ;
#11011=CARTESIAN_POINT ( 'NONE',  ( -154.9999999999999716, -23.00000000000000000, 10.00000000000000000 ) ) ;
#11034=VERTEX_POINT ( 'NONE', #9613 ) ;
#11076=EDGE_CURVE ( 'NONE', #5544, #5970, #1954, .T. ) ;
#11084=DIRECTION ( 'NONE',  ( 1.000000000000000000, 0.000000000000000000, 0.000000000000000000 ) ) ;
#11085=DIRECTION ( 'NONE',  ( 1.000000000000000000, 0.000000000000000000, 0.000000000000000000 ) ) ;
#11093=CARTESIAN_POINT ( 'NONE',  ( -54.99999999999996447, -14.99999999999998579, -10.00000000000000000 ) ) ;
#11130=ORIENTED_EDGE ( 'NONE', *, *, #10960, .F. ) ;
#11138=ORIENTED_EDGE ( 'NONE', *, *, #12551, .T. ) ;
#11156=CYLINDRICAL_SURFACE ( 'NONE', #6126, 4.000000000000003553 ) ;
#11172=EDGE_CURVE ( 'NONE', #13956, #8949, #2737, .T. ) ;
#11190=CYLINDRICAL_SURFACE ( 'NONE', #7141, 4.000000000000003553 ) ;
#11193=CARTESIAN_POINT ( 'NONE',  ( -54.99999999999996447, -22.99999999999998579, -10.00000000000000000 ) ) ;
#11212=EDGE_LOOP ( 'NONE', ( #11603, #15094, #17480, #19252 ) ) ;
#11249=DIRECTION ( 'NONE',  ( 0.000000000000000000, 0.000000000000000000, 1.000000000000000000 ) ) ;
#11262=CARTESIAN_POINT ( 'NONE',  ( -54.99999999999996447, -14.99999999999998579, -10.00000000000000178 ) ) ;
#11291=CARTESIAN_POINT ( 'NONE',  ( -54.99999999999996447, -6.999999999999985789, 10.00000000000000000 ) ) ;
#11296=DIRECTION ( 'NONE',  ( -0.000000000000000000, -0.000000000000000000, 1.000000000000000000 ) ) ;
#11355=DIRECTION ( 'NONE',  ( 0.000000000000000000, 0.000000000000000000, -1.000000000000000000 ) ) ;
#11371=CARTESIAN_POINT ( 'NONE',  ( -54.99999999999996447, -22.99999999999998579, 15.00000000000000000 ) ) ;
#11377=DIRECTION ( 'NONE',  ( 0.000000000000000000, 0.000000000000000000, 1.000000000000000000 ) ) ;
#11379=CIRCLE ( 'NONE', #11705, 8.000000000000007105 ) ;
#11467=AXIS2_PLACEMENT_3D ( 'NONE', #17967, #10484, #48 ) ;
#11498=CARTESIAN_POINT ( 'NONE',  ( -57.64999999999994884, -14.99999999999998579, 15.00000000000000000 ) ) ;
#11509=CARTESIAN_POINT ( 'NONE',  ( -150.9999999999999716, -14.99999999999999645, 15.00000000000000000 ) ) ;
#11603=ORIENTED_EDGE ( 'NONE', *, *, #1121, .F. ) ;
#11617=CARTESIAN_POINT ( 'NONE',  ( -99.99999999999997158, -23.00000000000000711, -15.00000000000000000 ) ) ;
#11677=CARTESIAN_POINT ( 'NONE',  ( -54.99999999999996447, -14.99999999999998579, -15.00000000000000000 ) ) ;
#11697=ORIENTED_EDGE ( 'NONE', *, *, #18659, .T. ) ;
#11705=AXIS2_PLACEMENT_3D ( 'NONE', #13063, #5810, #2784 ) ;
#11752=CARTESIAN_POINT ( 'NONE',  ( -150.9999999999999716, -14.99999999999999645, 15.00000000000000000 ) ) ;
#11768=CYLINDRICAL_SURFACE ( 'NONE', #5530, 2.649999999999985700 ) ;
#11776=CIRCLE ( 'NONE', #11467, 4.000000000000003553 ) ;
#11793=ORIENTED_EDGE ( 'NONE', *, *, #2450, .T. ) ;
#11808=DIRECTION ( 'NONE',  ( -1.000000000000000000, 0.000000000000000000, 0.000000000000000000 ) ) ;
#11835=AXIS2_PLACEMENT_3D ( 'NONE', #3340, #7929, #18256 ) ;
#11838=DIRECTION ( 'NONE',  ( -0.000000000000000000, -0.000000000000000000, 1.000000000000000000 ) ) ;
#11848=UNCERTAINTY_MEASURE_WITH_UNIT (LENGTH_MEASURE( 1.000000000000000082E-05 ), #9563, 'distance_accuracy_value', 'NONE');
#11881=ORIENTED_EDGE ( 'NONE', *, *, #4229, .T. ) ;
#11893=CARTESIAN_POINT ( 'NONE',  ( -162.9999999999999716, -14.99999999999999645, -15.00000000000000000 ) ) ;
#11899=AXIS2_PLACEMENT_3D ( 'NONE', #3448, #6758, #790 ) ;
#11958=AXIS2_PLACEMENT_3D ( 'NONE', #10160, #2832, #5856 ) ;
#11965=FACE_OUTER_BOUND ( 'NONE', #2218, .T. ) ;
#11982=CARTESIAN_POINT ( 'NONE',  ( -54.99999999999996447, -14.99999999999998579, -15.00000000000000000 ) ) ;
#11986=VERTEX_POINT ( 'NONE', #16519 ) ;
#12011=ORIENTED_EDGE ( 'NONE', *, *, #18080, .F. ) ;
#12030=DIRECTION ( 'NONE',  ( -0.000000000000000000, -0.000000000000000000, 1.000000000000000000 ) ) ;
#12036=DIRECTION ( 'NONE',  ( 1.000000000000000000, 0.000000000000000000, 0.000000000000000000 ) ) ;
#12037=VECTOR ( 'NONE', #18744, 1000.000000000000000 ) ;
#12056=AXIS2_PLACEMENT_3D ( 'NONE', #343, #4467, #16526 ) ;
#12086=ORIENTED_EDGE ( 'NONE', *, *, #5195, .F. ) ;
#12094=LINE ( 'NONE', #2003, #4643 ) ;
#12105=FACE_OUTER_BOUND ( 'NONE', #12682, .T. ) ;
#12127=ORIENTED_EDGE ( 'NONE', *, *, #19355, .T. ) ;
#12137=EDGE_LOOP ( 'NONE', ( #11130, #19011, #1265, #4308, #13391, #1536, #10336, #4654, #17005, #4645, #12186, #8681 ) ) ;
#12177=CARTESIAN_POINT ( 'NONE',  ( -54.99999999999996447, -14.99999999999998579, 15.00000000000000000 ) ) ;
#12186=ORIENTED_EDGE ( 'NONE', *, *, #82, .T. ) ;
#12202=EDGE_LOOP ( 'NONE', ( #10247, #1720 ) ) ;
#12235=VERTEX_POINT ( 'NONE', #12372 ) ;
#12257=ORIENTED_EDGE ( 'NONE', *, *, #4373, .F. ) ;
#12265=VECTOR ( 'NONE', #11296, 1000.000000000000000 ) ;
#12267=DIRECTION ( 'NONE',  ( 1.000000000000000000, 0.000000000000000000, 0.000000000000000000 ) ) ;
#12276=CARTESIAN_POINT ( 'NONE',  ( -54.99999999999996447, -14.99999999999998579, 10.00000000000000000 ) ) ;
#12291=FACE_BOUND ( 'NONE', #19129, .T. ) ;
#12298=ORIENTED_EDGE ( 'NONE', *, *, #3283, .F. ) ;
#12308=EDGE_LOOP ( 'NONE', ( #10339, #12927, #5930, #15219 ) ) ;
#12358=CARTESIAN_POINT ( 'NONE',  ( -54.99999999999996447, -22.99999999999998579, 15.00000000000000000 ) ) ;
#12372=CARTESIAN_POINT ( 'NONE',  ( -162.9999999999999716, -14.99999999999999645, -10.00000000000000000 ) ) ;
#12392=EDGE_CURVE ( 'NONE', #13823, #1569, #12748, .T. ) ;
#12393=DIRECTION ( 'NONE',  ( -1.000000000000000000, -1.387778780781445676E-16, 0.000000000000000000 ) ) ;
#12423=ORIENTED_EDGE ( 'NONE', *, *, #15912, .T. ) ;
#12427=UNCERTAINTY_MEASURE_WITH_UNIT (LENGTH_MEASURE( 1.000000000000000082E-05 ), #15851, 'distance_accuracy_value', 'NONE');
#12435=VECTOR ( 'NONE', #11355, 1000.000000000000000 ) ;
#12436=VERTEX_POINT ( 'NONE', #5712 ) ;
#12443=DIRECTION ( 'NONE',  ( 1.000000000000000000, 0.000000000000000000, 0.000000000000000000 ) ) ;
#12448=UNCERTAINTY_MEASURE_WITH_UNIT (LENGTH_MEASURE( 1.000000000000000082E-05 ), #5376, 'distance_accuracy_value', 'NONE');
#12457=DIRECTION ( 'NONE',  ( -0.000000000000000000, -0.000000000000000000, 1.000000000000000000 ) ) ;
#12459=AXIS2_PLACEMENT_3D ( 'NONE', #19130, #11838, #12036 ) ;
#12484=AXIS2_PLACEMENT_3D ( 'NONE', #8172, #5422, #15927 ) ;
#12518=ORIENTED_EDGE ( 'NONE', *, *, #10211, .F. ) ;
#12551=EDGE_CURVE ( 'NONE', #3254, #12436, #19231, .T. ) ;
#12569=CARTESIAN_POINT ( 'NONE',  ( -54.99999999999996447, -14.99999999999998579, -10.00000000000000000 ) ) ;
#12574=DIRECTION ( 'NONE',  ( -1.000000000000000000, -1.040834085586084257E-16, -0.000000000000000000 ) ) ;
#12582=DIRECTION ( 'NONE',  ( -0.000000000000000000, -0.000000000000000000, -1.000000000000000000 ) ) ;
#12604=LINE ( 'NONE', #845, #8792 ) ;
#12611=( NAMED_UNIT ( * ) SI_UNIT ( $, .STERADIAN. ) SOLID_ANGLE_UNIT ( ) );
#12616=ORIENTED_EDGE ( 'NONE', *, *, #11076, .T. ) ;
#12619=EDGE_CURVE ( 'NONE', #3254, #11034, #7146, .T. ) ;
#12625=CARTESIAN_POINT ( 'NONE',  ( -158.9999999999999716, -14.99999999999999645, -15.00000000000000000 ) ) ;
#12682=EDGE_LOOP ( 'NONE', ( #3629, #11881, #10914, #10759 ) ) ;
#12696=CIRCLE ( 'NONE', #16773, 8.000000000000007105 ) ;
#12709=( NAMED_UNIT ( * ) PLANE_ANGLE_UNIT ( ) SI_UNIT ( $, .RADIAN. ) );
#12748=CIRCLE ( 'NONE', #8360, 8.000000000000007105 ) ;
#12766=ADVANCED_FACE ( 'NONE', ( #15409, #1989 ), #6303, .F. ) ;
#12784=CARTESIAN_POINT ( 'NONE',  ( -150.9999999999999716, -14.99999999999999645, -15.00000000000000000 ) ) ;
#12831=VERTEX_POINT ( 'NONE', #11371 ) ;
#12861=VECTOR ( 'NONE', #12582, 1000.000000000000000 ) ;
#12871=FACE_OUTER_BOUND ( 'NONE', #13946, .T. ) ;
#12873=CARTESIAN_POINT ( 'NONE',  ( -162.9999999999999716, -14.99999999999999645, 15.00000000000000000 ) ) ;
#12884=ORIENTED_EDGE ( 'NONE', *, *, #2087, .T. ) ;
#12899=CIRCLE ( 'NONE', #11958, 4.000000000000003553 ) ;
#12927=ORIENTED_EDGE ( 'NONE', *, *, #5195, .T. ) ;
#12969=ORIENTED_EDGE ( 'NONE', *, *, #7876, .T. ) ;
#13009=CIRCLE ( 'NONE', #15204, 2.649999999999985700 ) ;
#13056=CARTESIAN_POINT ( 'NONE',  ( -154.9999999999999716, -14.99999999999999645, 15.00000000000000000 ) ) ;
#13061=LINE ( 'NONE', #11291, #15264 ) ;
#13063=CARTESIAN_POINT ( 'NONE',  ( -154.9999999999999716, -14.99999999999999645, -15.00000000000000000 ) ) ;
#13103=LINE ( 'NONE', #16060, #13337 ) ;
#13124=DIRECTION ( 'NONE',  ( -1.387778780781445676E-16, 1.000000000000000000, 0.000000000000000000 ) ) ;
#13144=DIRECTION ( 'NONE',  ( 1.000000000000000000, 0.000000000000000000, 0.000000000000000000 ) ) ;
#13154=AXIS2_PLACEMENT_3D ( 'NONE', #17759, #7353, #8017 ) ;
#13161=LINE ( 'NONE', #12873, #15462 ) ;
#13165=EDGE_CURVE ( 'NONE', #17750, #3558, #7779, .T. ) ;
#13177=CARTESIAN_POINT ( 'NONE',  ( -154.9999999999999716, -14.99999999999999645, 15.00000000000000000 ) ) ;
#13212=ADVANCED_FACE ( 'NONE', ( #11965 ), #8021, .F. ) ;
#13213=DIRECTION ( 'NONE',  ( -0.000000000000000000, -0.000000000000000000, 1.000000000000000000 ) ) ;
#13214=DIRECTION ( 'NONE',  ( 1.000000000000000000, 0.000000000000000000, 0.000000000000000000 ) ) ;
#13220=CARTESIAN_POINT ( 'NONE',  ( -54.99999999999996447, -6.999999999999985789, -10.00000000000000000 ) ) ;
#13261=ORIENTED_EDGE ( 'NONE', *, *, #13563, .T. ) ;
#13337=VECTOR ( 'NONE', #18820, 1000.000000000000000 ) ;
#13344=FACE_OUTER_BOUND ( 'NONE', #9542, .T. ) ;
#13391=ORIENTED_EDGE ( 'NONE', *, *, #1978, .T. ) ;
#13426=PRODUCT_DEFINITION_CONTEXT ( 'detailed design', #9646, 'design' ) ;
#13483=CARTESIAN_POINT ( 'NONE',  ( -154.9999999999999716, -14.99999999999999645, -10.00000000000000178 ) ) ;
#13489=VERTEX_POINT ( 'NONE', #8994 ) ;
#13498=ORIENTED_EDGE ( 'NONE', *, *, #10577, .T. ) ;
#13519=AXIS2_PLACEMENT_3D ( 'NONE', #9365, #6524, #7281 ) ;
#13521=EDGE_LOOP ( 'NONE', ( #16213, #11697 ) ) ;
#13563=EDGE_CURVE ( 'NONE', #730, #5970, #4659, .T. ) ;
#13574=DIRECTION ( 'NONE',  ( -0.000000000000000000, -0.000000000000000000, -1.000000000000000000 ) ) ;
#13603=ORIENTED_EDGE ( 'NONE', *, *, #82, .F. ) ;
#13604=CARTESIAN_POINT ( 'NONE',  ( -99.99999999999997158, -6.999999999999992895, 15.00000000000000000 ) ) ;
#13616=LINE ( 'NONE', #18342, #18723 ) ;
#13620=DIRECTION ( 'NONE',  ( 0.000000000000000000, 0.000000000000000000, 1.000000000000000000 ) ) ;
#13621=CARTESIAN_POINT ( 'NONE',  ( -54.99999999999996447, -22.99999999999998579, -15.00000000000000000 ) ) ;
#13639=CARTESIAN_POINT ( 'NONE',  ( -99.99999999999997158, -6.999999999999992895, 10.00000000000000000 ) ) ;
#13691=ORIENTED_EDGE ( 'NONE', *, *, #5191, .T. ) ;
#13705=EDGE_CURVE ( 'NONE', #402, #3962, #16850, .T. ) ;
#13723=ORIENTED_EDGE ( 'NONE', *, *, #4373, .T. ) ;
#13733=FACE_OUTER_BOUND ( 'NONE', #17318, .T. ) ;
#13763=DIRECTION ( 'NONE',  ( 1.000000000000000000, 0.000000000000000000, 0.000000000000000000 ) ) ;
#13768=VERTEX_POINT ( 'NONE', #3412 ) ;
#13823=VERTEX_POINT ( 'NONE', #9472 ) ;
#13920=DIRECTION ( 'NONE',  ( 0.000000000000000000, 0.000000000000000000, 1.000000000000000000 ) ) ;
#13934=CYLINDRICAL_SURFACE ( 'NONE', #10204, 8.000000000000007105 ) ;
#13946=EDGE_LOOP ( 'NONE', ( #187, #12884, #14615, #2516 ) ) ;
#13956=VERTEX_POINT ( 'NONE', #14472 ) ;
#13977=CARTESIAN_POINT ( 'NONE',  ( -158.9999999999999716, -14.99999999999999645, 10.00000000000000000 ) ) ;
#14004=ORIENTED_EDGE ( 'NONE', *, *, #1375, .T. ) ;
#14033=DIRECTION ( 'NONE',  ( -0.000000000000000000, -0.000000000000000000, 1.000000000000000000 ) ) ;
#14260=VECTOR ( 'NONE', #13213, 1000.000000000000000 ) ;
#14280=VECTOR ( 'NONE', #12574, 1000.000000000000000 ) ;
#14300=DIRECTION ( 'NONE',  ( -0.000000000000000000, -0.000000000000000000, 1.000000000000000000 ) ) ;
#14341=FACE_OUTER_BOUND ( 'NONE', #365, .T. ) ;
#14359=STYLED_ITEM ( 'NONE', ( #6531 ), #14807 ) ;
#14386=AXIS2_PLACEMENT_3D ( 'NONE', #13056, #2880, #17876 ) ;
#14431=VERTEX_POINT ( 'NONE', #12784 ) ;
#14437=ADVANCED_FACE ( 'NONE', ( #8070, #15828, #923 ), #629, .T. ) ;
#14443=CARTESIAN_POINT ( 'NONE',  ( -54.99999999999996447, -22.99999999999998579, 15.00000000000000000 ) ) ;
#14472=CARTESIAN_POINT ( 'NONE',  ( -154.9999999999999716, -23.00000000000000000, -15.00000000000000000 ) ) ;
#14488=PRODUCT_DEFINITION_FORMATION_WITH_SPECIFIED_SOURCE ( 'ANY', '', #16350, .NOT_KNOWN. ) ;
#14525=ADVANCED_FACE ( 'NONE', ( #14341 ), #729, .T. ) ;
#14542=ORIENTED_EDGE ( 'NONE', *, *, #19355, .F. ) ;
#14615=ORIENTED_EDGE ( 'NONE', *, *, #19061, .F. ) ;
#14618=DIRECTION ( 'NONE',  ( 1.000000000000000000, 0.000000000000000000, 0.000000000000000000 ) ) ;
#14637=AXIS2_PLACEMENT_3D ( 'NONE', #11093, #14033, #519 ) ;
#14649=LINE ( 'NONE', #15053, #1263 ) ;
#14701=AXIS2_PLACEMENT_3D ( 'NONE', #608, #11377, #2389 ) ;
#14717=AXIS2_PLACEMENT_3D ( 'NONE', #8919, #1379, #17861 ) ;
#14792=EDGE_LOOP ( 'NONE', ( #12011, #1966 ) ) ;
#14807=ADVANCED_BREP_SHAPE_REPRESENTATION ( '', ( #2264, #10359 ), #3416 ) ;
#14843=FACE_OUTER_BOUND ( 'NONE', #6848, .T. ) ;
#14846=VECTOR ( 'NONE', #2194, 1000.000000000000000 ) ;
#14847=DIRECTION ( 'NONE',  ( 1.000000000000000000, 1.387778780781445676E-16, 0.000000000000000000 ) ) ;
#14868=CIRCLE ( 'NONE', #3286, 4.000000000000003553 ) ;
#14947=CARTESIAN_POINT ( 'NONE',  ( -154.9999999999999716, -23.00000000000000000, 15.00000000000000000 ) ) ;
#15018=CARTESIAN_POINT ( 'NONE',  ( -54.99999999999996447, -14.99999999999998579, -15.00000000000000000 ) ) ;
#15029=EDGE_CURVE ( 'NONE', #402, #4701, #4405, .T. ) ;
#15053=CARTESIAN_POINT ( 'NONE',  ( -154.9999999999999716, -6.999999999999993783, 15.00000000000000000 ) ) ;
#15077=DIRECTION ( 'NONE',  ( 1.000000000000000000, 1.387778780781445676E-16, 0.000000000000000000 ) ) ;
#15094=ORIENTED_EDGE ( 'NONE', *, *, #1978, .F. ) ;
#15119=CARTESIAN_POINT ( 'NONE',  ( -57.64999999999994884, -14.99999999999998579, 10.00000000000000000 ) ) ;
#15204=AXIS2_PLACEMENT_3D ( 'NONE', #5777, #17748, #5681 ) ;
#15219=ORIENTED_EDGE ( 'NONE', *, *, #17077, .F. ) ;
#15264=VECTOR ( 'NONE', #7179, 1000.000000000000000 ) ;
#15281=CARTESIAN_POINT ( 'NONE',  ( -52.34999999999998010, -14.99999999999998579, 10.00000000000000000 ) ) ;
#15293=ORIENTED_EDGE ( 'NONE', *, *, #15912, .F. ) ;
#15360=AXIS2_PLACEMENT_3D ( 'NONE', #507, #12457, #18469 ) ;
#15378=DIRECTION ( 'NONE',  ( -1.000000000000000000, -1.387778780781445182E-16, -0.000000000000000000 ) ) ;
#15389=VERTEX_POINT ( 'NONE', #18816 ) ;
#15409=FACE_BOUND ( 'NONE', #12202, .T. ) ;
#15462=VECTOR ( 'NONE', #1019, 1000.000000000000000 ) ;
#15474=AXIS2_PLACEMENT_3D ( 'NONE', #6468, #6294, #12267 ) ;
#15482=ORIENTED_EDGE ( 'NONE', *, *, #15029, .T. ) ;
#15491=DIRECTION ( 'NONE',  ( 1.000000000000000000, 0.000000000000000000, 0.000000000000000000 ) ) ;
#15503=FACE_OUTER_BOUND ( 'NONE', #2385, .T. ) ;
#15506=DIRECTION ( 'NONE',  ( 0.000000000000000000, 0.000000000000000000, 1.000000000000000000 ) ) ;
#15566=CARTESIAN_POINT ( 'NONE',  ( -150.9999999999999716, -14.99999999999999645, 15.00000000000000000 ) ) ;
#15589=AXIS2_PLACEMENT_3D ( 'NONE', #17011, #617, #718 ) ;
#15601=VECTOR ( 'NONE', #5775, 1000.000000000000000 ) ;
#15613=LINE ( 'NONE', #515, #14280 ) ;
#15634=AXIS2_PLACEMENT_3D ( 'NONE', #6896, #6702, #5135 ) ;
#15641=ORIENTED_EDGE ( 'NONE', *, *, #11076, .F. ) ;
#15655=ORIENTED_EDGE ( 'NONE', *, *, #7350, .T. ) ;
#15674=CARTESIAN_POINT ( 'NONE',  ( -54.99999999999996447, -6.999999999999985789, -10.00000000000000000 ) ) ;
#15696=DIRECTION ( 'NONE',  ( 0.000000000000000000, 0.000000000000000000, -1.000000000000000000 ) ) ;
#15697=VECTOR ( 'NONE', #16253, 1000.000000000000000 ) ;
#15744=ADVANCED_FACE ( 'NONE', ( #12105 ), #4859, .T. ) ;
#15807=DIRECTION ( 'NONE',  ( 0.000000000000000000, 0.000000000000000000, -1.000000000000000000 ) ) ;
#15827=EDGE_LOOP ( 'NONE', ( #7916, #9406, #36, #7895 ) ) ;
#15828=FACE_OUTER_BOUND ( 'NONE', #17286, .T. ) ;
#15829=ORIENTED_EDGE ( 'NONE', *, *, #5984, .T. ) ;
#15851=( LENGTH_UNIT ( ) NAMED_UNIT ( * ) SI_UNIT ( .MILLI., .METRE. ) );
#15912=EDGE_CURVE ( 'NONE', #12436, #2611, #18688, .T. ) ;
#15927=DIRECTION ( 'NONE',  ( 1.000000000000000000, 0.000000000000000000, -0.000000000000000000 ) ) ;
#15960=ORIENTED_EDGE ( 'NONE', *, *, #15029, .F. ) ;
#15979=VECTOR ( 'NONE', #8585, 1000.000000000000000 ) ;
#15991=CIRCLE ( 'NONE', #14717, 2.649999999999985700 ) ;
#15999=CIRCLE ( 'NONE', #5664, 8.000000000000007105 ) ;
#16060=CARTESIAN_POINT ( 'NONE',  ( -52.34999999999998010, -14.99999999999998579, 15.00000000000000000 ) ) ;
#16120=EDGE_CURVE ( 'NONE', #9930, #730, #330, .T. ) ;
#16123=ORIENTED_EDGE ( 'NONE', *, *, #7171, .T. ) ;
#16191=DIRECTION ( 'NONE',  ( 1.000000000000000000, 0.000000000000000000, 0.000000000000000000 ) ) ;
#16193=VERTEX_POINT ( 'NONE', #7578 ) ;
#16213=ORIENTED_EDGE ( 'NONE', *, *, #1257, .T. ) ;
#16252=MECHANICAL_DESIGN_GEOMETRIC_PRESENTATION_REPRESENTATION('',(#14359),#5915);
#16253=DIRECTION ( 'NONE',  ( -0.000000000000000000, -0.000000000000000000, 1.000000000000000000 ) ) ;
#16263=VECTOR ( 'NONE', #6348, 1000.000000000000000 ) ;
#16287=EDGE_CURVE ( 'NONE', #12831, #10827, #3748, .T. ) ;
#16295=DIRECTION ( 'NONE',  ( 1.000000000000000000, 0.000000000000000000, 0.000000000000000000 ) ) ;
#16300=ADVANCED_FACE ( 'NONE', ( #9808, #6583 ), #6778, .F. ) ;
#16350=PRODUCT ( 'reel holder bar', 'reel holder bar', '', ( #17766 ) ) ;
#16395=DIRECTION ( 'NONE',  ( -0.000000000000000000, -0.000000000000000000, 1.000000000000000000 ) ) ;
#16405=CARTESIAN_POINT ( 'NONE',  ( -162.9999999999999716, -14.99999999999999645, 15.00000000000000000 ) ) ;
#16412=CARTESIAN_POINT ( 'NONE',  ( -154.9999999999999716, -14.99999999999999645, -10.00000000000000000 ) ) ;
#16457=CARTESIAN_POINT ( 'NONE',  ( -158.9999999999999716, -14.99999999999999645, -10.00000000000000178 ) ) ;
#16519=CARTESIAN_POINT ( 'NONE',  ( -150.9999999999999716, -14.99999999999999645, -10.00000000000000178 ) ) ;
#16526=DIRECTION ( 'NONE',  ( -1.000000000000000000, 0.000000000000000000, -0.000000000000000000 ) ) ;
#16555=LINE ( 'NONE', #17939, #14260 ) ;
#16636=AXIS2_PLACEMENT_3D ( 'NONE', #12177, #16704, #6383 ) ;
#16651=AXIS2_PLACEMENT_3D ( 'NONE', #13483, #5838, #11808 ) ;
#16704=DIRECTION ( 'NONE',  ( -0.000000000000000000, -0.000000000000000000, 1.000000000000000000 ) ) ;
#16766=AXIS2_PLACEMENT_3D ( 'NONE', #6, #13620, #4610 ) ;
#16773=AXIS2_PLACEMENT_3D ( 'NONE', #2064, #8026, #12443 ) ;
#16785=DIRECTION ( 'NONE',  ( -0.000000000000000000, -0.000000000000000000, 1.000000000000000000 ) ) ;
#16787=PLANE ( 'NONE',  #15474 ) ;
#16823=EDGE_LOOP ( 'NONE', ( #7123, #19358, #5064, #3964 ) ) ;
#16850=LINE ( 'NONE', #13604, #16263 ) ;
#16948=( NAMED_UNIT ( * ) SI_UNIT ( $, .STERADIAN. ) SOLID_ANGLE_UNIT ( ) );
#16954=ORIENTED_EDGE ( 'NONE', *, *, #7876, .F. ) ;
#16990=DIRECTION ( 'NONE',  ( -0.000000000000000000, -0.000000000000000000, 1.000000000000000000 ) ) ;
#17005=ORIENTED_EDGE ( 'NONE', *, *, #7171, .F. ) ;
#17011=CARTESIAN_POINT ( 'NONE',  ( -54.99999999999996447, -14.99999999999998579, 15.00000000000000000 ) ) ;
#17069=ADVANCED_FACE ( 'NONE', ( #1490 ), #4819, .F. ) ;
#17077=EDGE_CURVE ( 'NONE', #12235, #8949, #3151, .T. ) ;
#17101=DIRECTION ( 'NONE',  ( 1.000000000000000000, 0.000000000000000000, 0.000000000000000000 ) ) ;
#17110=VECTOR ( 'NONE', #10573, 1000.000000000000000 ) ;
#17116=VERTEX_POINT ( 'NONE', #18652 ) ;
#17137=SURFACE_STYLE_USAGE ( .BOTH. , #3895 ) ;
#17216=DIRECTION ( 'NONE',  ( -0.000000000000000000, -0.000000000000000000, 1.000000000000000000 ) ) ;
#17241=ORIENTED_EDGE ( 'NONE', *, *, #6675, .T. ) ;
#17273=CARTESIAN_POINT ( 'NONE',  ( -99.99999999999997158, -6.999999999999989342, -10.00000000000000000 ) ) ;
#17286=EDGE_LOOP ( 'NONE', ( #13498, #5358, #13723, #17564, #1143 ) ) ;
#17318=EDGE_LOOP ( 'NONE', ( #18033, #8564, #18246, #12518 ) ) ;
#17337=ORIENTED_EDGE ( 'NONE', *, *, #2329, .F. ) ;
#17339=FILL_AREA_STYLE ('',( #2336 ) ) ;
#17354=PLANE ( 'NONE',  #962 ) ;
#17404=ORIENTED_EDGE ( 'NONE', *, *, #10577, .F. ) ;
#17413=ORIENTED_EDGE ( 'NONE', *, *, #8072, .T. ) ;
#17448=( NAMED_UNIT ( * ) PLANE_ANGLE_UNIT ( ) SI_UNIT ( $, .RADIAN. ) );
#17461=CARTESIAN_POINT ( 'NONE',  ( -54.99999999999996447, -6.999999999999985789, 10.00000000000000000 ) ) ;
#17480=ORIENTED_EDGE ( 'NONE', *, *, #1495, .T. ) ;
#17544=CARTESIAN_POINT ( 'NONE',  ( -154.9999999999999716, -6.999999999999993783, -10.00000000000000000 ) ) ;
#17564=ORIENTED_EDGE ( 'NONE', *, *, #19255, .T. ) ;
#17565=EDGE_LOOP ( 'NONE', ( #13691, #2988, #8442, #16123 ) ) ;
#17595=FACE_OUTER_BOUND ( 'NONE', #12308, .T. ) ;
#17627=CARTESIAN_POINT ( 'NONE',  ( -54.99999999999996447, -22.99999999999998579, -15.00000000000000000 ) ) ;
#17647=DIRECTION ( 'NONE',  ( -0.000000000000000000, -0.000000000000000000, 1.000000000000000000 ) ) ;
#17680=DIRECTION ( 'NONE',  ( 1.000000000000000000, 0.000000000000000000, 0.000000000000000000 ) ) ;
#17681=DIRECTION ( 'NONE',  ( 0.000000000000000000, 0.000000000000000000, 1.000000000000000000 ) ) ;
#17682=LINE ( 'NONE', #4334, #4612 ) ;
#17721=CARTESIAN_POINT ( 'NONE',  ( -154.9999999999999716, -23.00000000000000000, -10.00000000000000000 ) ) ;
#17748=DIRECTION ( 'NONE',  ( 0.000000000000000000, 0.000000000000000000, -1.000000000000000000 ) ) ;
#17750=VERTEX_POINT ( 'NONE', #1902 ) ;
#17759=CARTESIAN_POINT ( 'NONE',  ( -154.9999999999999716, -14.99999999999999645, 10.00000000000000000 ) ) ;
#17766=PRODUCT_CONTEXT ( 'NONE', #17808, 'mechanical' ) ;
#17769=CLOSED_SHELL ( 'NONE', ( #17069, #4132, #1270, #18041, #9395, #3431, #14525, #15744, #6278, #1157, #13212, #7656, #5667, #14437, #12766, #1069, #8796, #10815, #3738, #4009, #16300, #4954, #105, #19154 ) ) ;
#17774=CARTESIAN_POINT ( 'NONE',  ( -54.99999999999996447, -14.99999999999998579, 15.00000000000000000 ) ) ;
#17786=VERTEX_POINT ( 'NONE', #3850 ) ;
#17796=ORIENTED_EDGE ( 'NONE', *, *, #10211, .T. ) ;
#17808=APPLICATION_CONTEXT ( 'automotive_design' ) ;
#17861=DIRECTION ( 'NONE',  ( 1.000000000000000000, 0.000000000000000000, 0.000000000000000000 ) ) ;
#17876=DIRECTION ( 'NONE',  ( 1.000000000000000000, 0.000000000000000000, 0.000000000000000000 ) ) ;
#17877=CIRCLE ( 'NONE', #13154, 8.000000000000007105 ) ;
#17900=ORIENTED_EDGE ( 'NONE', *, *, #7350, .F. ) ;
#17939=CARTESIAN_POINT ( 'NONE',  ( -54.99999999999996447, -6.999999999999985789, -15.00000000000000000 ) ) ;
#17967=CARTESIAN_POINT ( 'NONE',  ( -154.9999999999999716, -14.99999999999999645, -15.00000000000000000 ) ) ;
#18008=CARTESIAN_POINT ( 'NONE',  ( -54.99999999999996447, -22.99999999999998579, 10.00000000000000000 ) ) ;
#18033=ORIENTED_EDGE ( 'NONE', *, *, #13165, .F. ) ;
#18041=ADVANCED_FACE ( 'NONE', ( #1102 ), #2597, .F. ) ;
#18047=EDGE_CURVE ( 'NONE', #3558, #17750, #5950, .T. ) ;
#18080=EDGE_CURVE ( 'NONE', #5970, #730, #10939, .T. ) ;
#18089=VECTOR ( 'NONE', #6647, 1000.000000000000000 ) ;
#18100=FACE_OUTER_BOUND ( 'NONE', #7342, .T. ) ;
#18144=ORIENTED_EDGE ( 'NONE', *, *, #5937, .T. ) ;
#18184=AXIS2_PLACEMENT_3D ( 'NONE', #2104, #9343, #13763 ) ;
#18208=VECTOR ( 'NONE', #3187, 1000.000000000000000 ) ;
#18217=DIRECTION ( 'NONE',  ( -1.000000000000000000, -1.040834085586084257E-16, 0.000000000000000000 ) ) ;
#18244=ORIENTED_EDGE ( 'NONE', *, *, #18659, .F. ) ;
#18246=ORIENTED_EDGE ( 'NONE', *, *, #347, .F. ) ;
#18251=LINE ( 'NONE', #1866, #2061 ) ;
#18256=DIRECTION ( 'NONE',  ( 1.000000000000000000, 1.040834085586084257E-16, 0.000000000000000000 ) ) ;
#18289=LINE ( 'NONE', #2094, #14846 ) ;
#18307=CARTESIAN_POINT ( 'NONE',  ( -54.99999999999996447, -6.999999999999985789, 15.00000000000000000 ) ) ;
#18325=VERTEX_POINT ( 'NONE', #17627 ) ;
#18342=CARTESIAN_POINT ( 'NONE',  ( -99.99999999999997158, -6.999999999999992895, -15.00000000000000000 ) ) ;
#18352=EDGE_CURVE ( 'NONE', #18325, #13956, #7112, .T. ) ;
#18360=FACE_OUTER_BOUND ( 'NONE', #4941, .T. ) ;
#18387=FACE_OUTER_BOUND ( 'NONE', #6705, .T. ) ;
#18469=DIRECTION ( 'NONE',  ( 1.000000000000000000, 0.000000000000000000, 0.000000000000000000 ) ) ;
#18479=CARTESIAN_POINT ( 'NONE',  ( -154.9999999999999716, -14.99999999999999645, 15.00000000000000000 ) ) ;
#18483=FACE_OUTER_BOUND ( 'NONE', #17565, .T. ) ;
#18548=AXIS2_PLACEMENT_3D ( 'NONE', #12358, #10885, #701 ) ;
#18551=ORIENTED_EDGE ( 'NONE', *, *, #9565, .T. ) ;
#18569=EDGE_CURVE ( 'NONE', #3254, #13489, #10625, .T. ) ;
#18583=CARTESIAN_POINT ( 'NONE',  ( -52.34999999999998010, -14.99999999999998579, -15.00000000000000000 ) ) ;
#18623=VERTEX_POINT ( 'NONE', #7595 ) ;
#18632=EDGE_CURVE ( 'NONE', #13823, #17116, #14649, .T. ) ;
#18652=CARTESIAN_POINT ( 'NONE',  ( -154.9999999999999716, -6.999999999999993783, 10.00000000000000000 ) ) ;
#18659=EDGE_CURVE ( 'NONE', #5389, #7908, #2537, .T. ) ;
#18688=LINE ( 'NONE', #9738, #9048 ) ;
#18723=VECTOR ( 'NONE', #15378, 1000.000000000000000 ) ;
#18729=CIRCLE ( 'NONE', #10877, 8.000000000000000000 ) ;
#18744=DIRECTION ( 'NONE',  ( 1.387778780781445676E-16, -1.000000000000000000, 0.000000000000000000 ) ) ;
#18812=( NAMED_UNIT ( * ) PLANE_ANGLE_UNIT ( ) SI_UNIT ( $, .RADIAN. ) );
#18816=CARTESIAN_POINT ( 'NONE',  ( -52.34999999999998010, -14.99999999999998579, 15.00000000000000178 ) ) ;
#18820=DIRECTION ( 'NONE',  ( -0.000000000000000000, -0.000000000000000000, 1.000000000000000000 ) ) ;
#18910=VERTEX_POINT ( 'NONE', #5325 ) ;
#19011=ORIENTED_EDGE ( 'NONE', *, *, #5020, .F. ) ;
#19061=EDGE_CURVE ( 'NONE', #4701, #12235, #15999, .T. ) ;
#19068=DIRECTION ( 'NONE',  ( -0.000000000000000000, -0.000000000000000000, 1.000000000000000000 ) ) ;
#19101=VECTOR ( 'NONE', #6390, 1000.000000000000000 ) ;
#19117=ORIENTED_EDGE ( 'NONE', *, *, #2519, .F. ) ;
#19129=EDGE_LOOP ( 'NONE', ( #7312, #19414 ) ) ;
#19130=CARTESIAN_POINT ( 'NONE',  ( -154.9999999999999716, -14.99999999999999645, 15.00000000000000000 ) ) ;
#19133=CARTESIAN_POINT ( 'NONE',  ( -74.99999999999997158, -23.00000000000000355, 15.00000000000000000 ) ) ;
#19152=AXIS2_PLACEMENT_3D ( 'NONE', #13177, #1324, #6116 ) ;
#19154=ADVANCED_FACE ( 'NONE', ( #15503 ), #4920, .F. ) ;
#19170=DIRECTION ( 'NONE',  ( 1.000000000000000000, 0.000000000000000000, 0.000000000000000000 ) ) ;
#19219=ORIENTED_EDGE ( 'NONE', *, *, #17077, .T. ) ;
#19231=LINE ( 'NONE', #19133, #12435 ) ;
#19233=DIRECTION ( 'NONE',  ( -1.000000000000000000, -1.040834085586084257E-16, 0.000000000000000000 ) ) ;
#19252=ORIENTED_EDGE ( 'NONE', *, *, #2329, .T. ) ;
#19253=CARTESIAN_POINT ( 'NONE',  ( -54.99999999999996447, -14.99999999999998579, -15.00000000000000000 ) ) ;
#19255=EDGE_CURVE ( 'NONE', #6843, #12831, #9513, .T. ) ;
#19296=DIRECTION ( 'NONE',  ( -0.000000000000000000, -0.000000000000000000, 1.000000000000000000 ) ) ;
#19355=EDGE_CURVE ( 'NONE', #15389, #16193, #7846, .T. ) ;
#19358=ORIENTED_EDGE ( 'NONE', *, *, #6450, .F. ) ;
#19414=ORIENTED_EDGE ( 'NONE', *, *, #13165, .T. ) ;
#19448=COLOUR_RGB('Light Blue',0.38,0.62,0.78);
#19449=FILL_AREA_STYLE_COLOUR('',#19448);
#19450=FILL_AREA_STYLE('',(#19449));
#19451=SURFACE_STYLE_FILL_AREA(#19450);
#19452=SURFACE_SIDE_STYLE('',(#19451));
#19453=SURFACE_STYLE_USAGE(.BOTH.,#19452);
#19454=PRESENTATION_STYLE_ASSIGNMENT((#19453));
ENDSEC;
END-ISO-10303-21;
